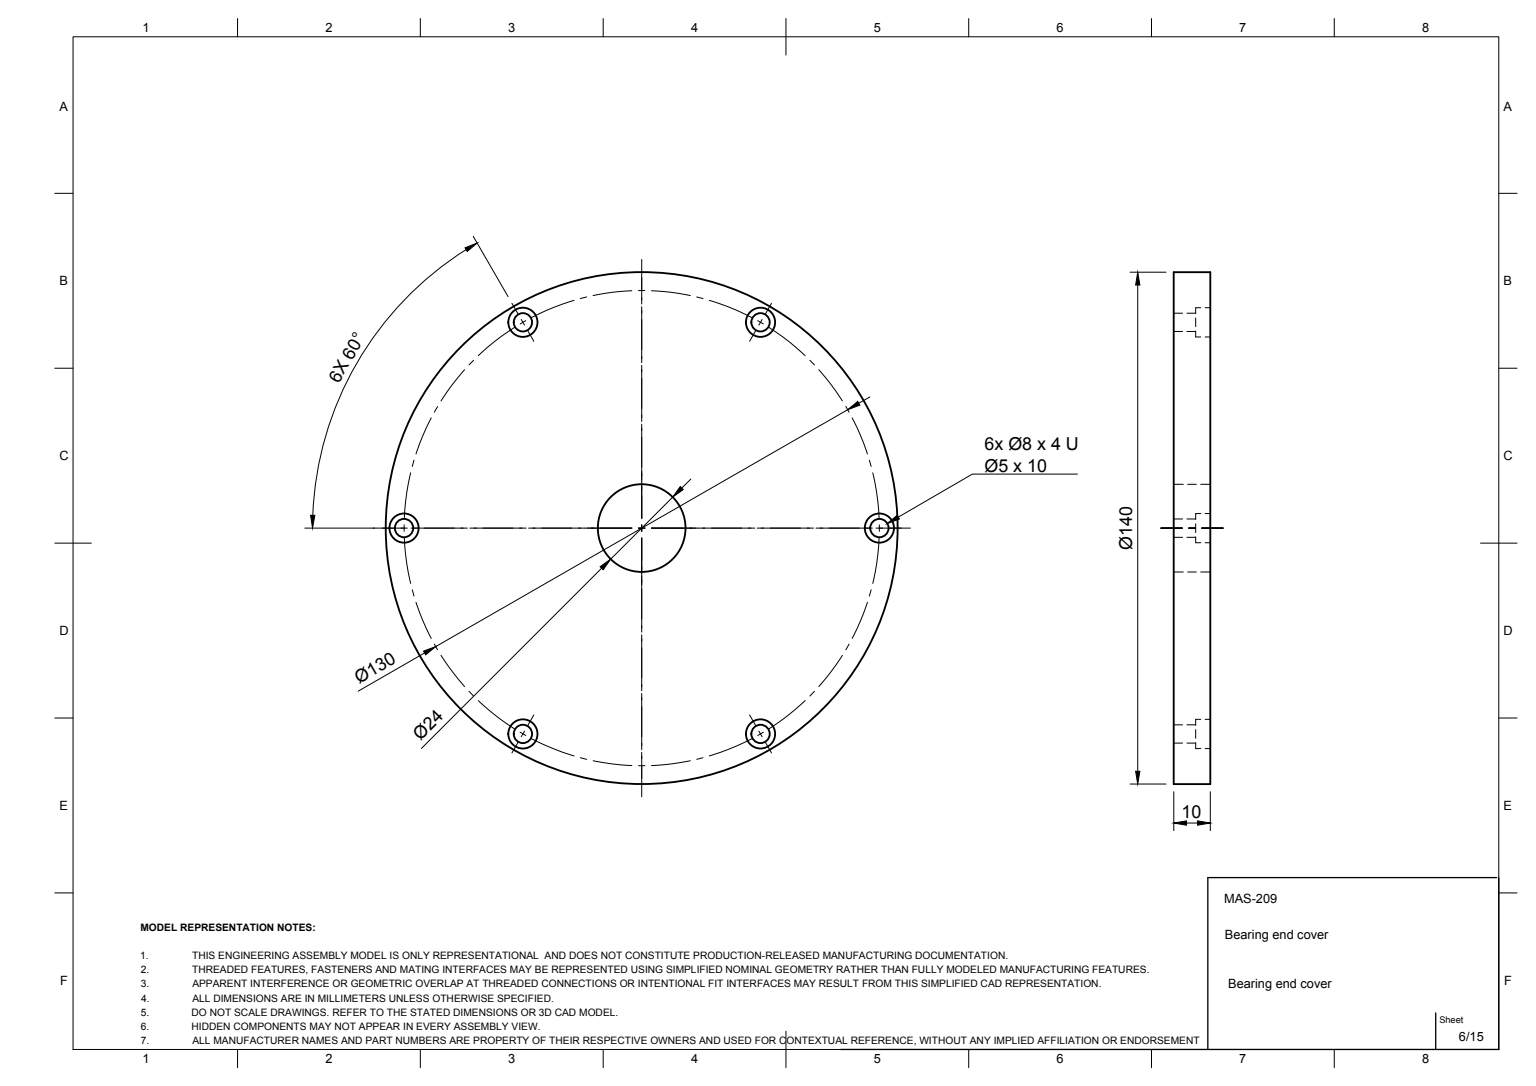
ISO-10303-21;
HEADER;
/* Generated by software containing ST-Developer
 * from STEP Tools, Inc. (www.steptools.com) 
 */

FILE_DESCRIPTION(
/* description */ ('Independent bearing-supported roller-ramp one-way clutch. Six logarit
hmic ramps with plain solid rollers, sprung guided plungers, native Co
il variants, removable shared keepers, rounded parallel key, shaft wit
h complete retaining lips, bronze journal/thrust support and bolted co
vers. Native rotor, roller planar/spin and plunger joints permit manua
l geometric engaged/released inspection. Automatic frictional torque s
witching/contact dynamics are not simulated; no capacity, hardness, fi
t, lubrication, speed, force or life rating. External input driver/cou
pling/anchors outside assembly.'),
/* implementation_level */ '2;1');

FILE_NAME(
/* name */ 'Bearing end cover.step',
/* time_stamp */ '2026-11-08T07:04:38-08:00',
/* author */ (''),
/* organization */ (''),
/* preprocessor_version */ 'ST-DEVELOPER v20.2',
/* originating_system */ 'Autodesk Translation Framework v15.17.0.0',
/* authorisation */ '');

FILE_SCHEMA (('AUTOMOTIVE_DESIGN { 1 0 10303 214 3 1 1 }'));
ENDSEC;

DATA;
#10=MECHANICAL_DESIGN_GEOMETRIC_PRESENTATION_REPRESENTATION('',(#305),#99526);
#273=SHAPE_REPRESENTATION_RELATIONSHIP('SRR','None',#99630,#289);
#289=ADVANCED_BREP_SHAPE_REPRESENTATION('',(#321),#99515);
#305=STYLED_ITEM('',(#99719),#321);
#321=MANIFOLD_SOLID_BREP('Body1',#18275);
#394=FACE_BOUND('',#2584,.T.);
#395=FACE_BOUND('',#2588,.T.);
#396=FACE_BOUND('',#2592,.T.);
#397=FACE_BOUND('',#2596,.T.);
#398=FACE_BOUND('',#2600,.T.);
#399=FACE_BOUND('',#2604,.T.);
#400=FACE_BOUND('',#2610,.T.);
#401=FACE_BOUND('',#2611,.T.);
#402=FACE_BOUND('',#2612,.T.);
#403=FACE_BOUND('',#2613,.T.);
#404=FACE_BOUND('',#2614,.T.);
#405=FACE_BOUND('',#2615,.T.);
#406=FACE_BOUND('',#2616,.T.);
#407=FACE_BOUND('',#2618,.T.);
#408=FACE_BOUND('',#2619,.T.);
#409=FACE_BOUND('',#2620,.T.);
#410=FACE_BOUND('',#2621,.T.);
#411=FACE_BOUND('',#2622,.T.);
#412=FACE_BOUND('',#2623,.T.);
#413=FACE_BOUND('',#2624,.T.);
#567=PLANE('',#19496);
#568=PLANE('',#19503);
#569=PLANE('',#19510);
#570=PLANE('',#19517);
#571=PLANE('',#19524);
#572=PLANE('',#19531);
#573=PLANE('',#19544);
#574=PLANE('',#19545);
#1524=FACE_OUTER_BOUND('',#2583,.T.);
#1525=FACE_OUTER_BOUND('',#2585,.T.);
#1526=FACE_OUTER_BOUND('',#2586,.T.);
#1527=FACE_OUTER_BOUND('',#2587,.T.);
#1528=FACE_OUTER_BOUND('',#2589,.T.);
#1529=FACE_OUTER_BOUND('',#2590,.T.);
#1530=FACE_OUTER_BOUND('',#2591,.T.);
#1531=FACE_OUTER_BOUND('',#2593,.T.);
#1532=FACE_OUTER_BOUND('',#2594,.T.);
#1533=FACE_OUTER_BOUND('',#2595,.T.);
#1534=FACE_OUTER_BOUND('',#2597,.T.);
#1535=FACE_OUTER_BOUND('',#2598,.T.);
#1536=FACE_OUTER_BOUND('',#2599,.T.);
#1537=FACE_OUTER_BOUND('',#2601,.T.);
#1538=FACE_OUTER_BOUND('',#2602,.T.);
#1539=FACE_OUTER_BOUND('',#2603,.T.);
#1540=FACE_OUTER_BOUND('',#2605,.T.);
#1541=FACE_OUTER_BOUND('',#2606,.T.);
#1542=FACE_OUTER_BOUND('',#2607,.T.);
#1543=FACE_OUTER_BOUND('',#2608,.T.);
#1544=FACE_OUTER_BOUND('',#2609,.T.);
#1545=FACE_OUTER_BOUND('',#2617,.T.);
#2583=EDGE_LOOP('',(#15852));
#2584=EDGE_LOOP('',(#15853));
#2585=EDGE_LOOP('',(#15854,#15855,#15856,#15857));
#2586=EDGE_LOOP('',(#15858,#15859,#15860,#15861));
#2587=EDGE_LOOP('',(#15862));
#2588=EDGE_LOOP('',(#15863));
#2589=EDGE_LOOP('',(#15864,#15865,#15866,#15867));
#2590=EDGE_LOOP('',(#15868,#15869,#15870,#15871));
#2591=EDGE_LOOP('',(#15872));
#2592=EDGE_LOOP('',(#15873));
#2593=EDGE_LOOP('',(#15874,#15875,#15876,#15877));
#2594=EDGE_LOOP('',(#15878,#15879,#15880,#15881));
#2595=EDGE_LOOP('',(#15882));
#2596=EDGE_LOOP('',(#15883));
#2597=EDGE_LOOP('',(#15884,#15885,#15886,#15887));
#2598=EDGE_LOOP('',(#15888,#15889,#15890,#15891));
#2599=EDGE_LOOP('',(#15892));
#2600=EDGE_LOOP('',(#15893));
#2601=EDGE_LOOP('',(#15894,#15895,#15896,#15897));
#2602=EDGE_LOOP('',(#15898,#15899,#15900,#15901));
#2603=EDGE_LOOP('',(#15902));
#2604=EDGE_LOOP('',(#15903));
#2605=EDGE_LOOP('',(#15904,#15905,#15906,#15907));
#2606=EDGE_LOOP('',(#15908,#15909,#15910,#15911));
#2607=EDGE_LOOP('',(#15912,#15913,#15914,#15915));
#2608=EDGE_LOOP('',(#15916,#15917,#15918,#15919));
#2609=EDGE_LOOP('',(#15920));
#2610=EDGE_LOOP('',(#15921));
#2611=EDGE_LOOP('',(#15922));
#2612=EDGE_LOOP('',(#15923));
#2613=EDGE_LOOP('',(#15924));
#2614=EDGE_LOOP('',(#15925));
#2615=EDGE_LOOP('',(#15926));
#2616=EDGE_LOOP('',(#15927));
#2617=EDGE_LOOP('',(#15928));
#2618=EDGE_LOOP('',(#15929));
#2619=EDGE_LOOP('',(#15930));
#2620=EDGE_LOOP('',(#15931));
#2621=EDGE_LOOP('',(#15932));
#2622=EDGE_LOOP('',(#15933));
#2623=EDGE_LOOP('',(#15934));
#2624=EDGE_LOOP('',(#15935));
#3022=CIRCLE('',#19497,4.);
#3023=CIRCLE('',#19498,2.5);
#3024=CIRCLE('',#19500,4.);
#3025=CIRCLE('',#19502,2.5);
#3026=CIRCLE('',#19504,4.);
#3027=CIRCLE('',#19505,2.5);
#3028=CIRCLE('',#19507,4.);
#3029=CIRCLE('',#19509,2.5);
#3030=CIRCLE('',#19511,4.);
#3031=CIRCLE('',#19512,2.5);
#3032=CIRCLE('',#19514,4.);
#3033=CIRCLE('',#19516,2.5);
#3034=CIRCLE('',#19518,4.);
#3035=CIRCLE('',#19519,2.5);
#3036=CIRCLE('',#19521,4.);
#3037=CIRCLE('',#19523,2.5);
#3038=CIRCLE('',#19525,4.);
#3039=CIRCLE('',#19526,2.5);
#3040=CIRCLE('',#19528,4.);
#3041=CIRCLE('',#19530,2.5);
#3042=CIRCLE('',#19532,4.);
#3043=CIRCLE('',#19533,2.5);
#3044=CIRCLE('',#19535,4.);
#3045=CIRCLE('',#19537,2.5);
#3046=CIRCLE('',#19539,12.);
#3047=CIRCLE('',#19540,12.);
#3048=CIRCLE('',#19542,70.);
#3049=CIRCLE('',#19543,70.);
#5400=LINE('',#94675,#6304);
#5401=LINE('',#94678,#6305);
#5402=LINE('',#94688,#6306);
#5403=LINE('',#94691,#6307);
#5404=LINE('',#94701,#6308);
#5405=LINE('',#94704,#6309);
#5406=LINE('',#94714,#6310);
#5407=LINE('',#94717,#6311);
#5408=LINE('',#94727,#6312);
#5409=LINE('',#94730,#6313);
#5410=LINE('',#94740,#6314);
#5411=LINE('',#94743,#6315);
#5412=LINE('',#94749,#6316);
#5413=LINE('',#94755,#6317);
#6304=VECTOR('',#22645,4.);
#6305=VECTOR('',#22648,2.5);
#6306=VECTOR('',#22661,4.);
#6307=VECTOR('',#22664,2.5);
#6308=VECTOR('',#22677,4.);
#6309=VECTOR('',#22680,2.5);
#6310=VECTOR('',#22693,4.);
#6311=VECTOR('',#22696,2.5);
#6312=VECTOR('',#22709,4.);
#6313=VECTOR('',#22712,2.5);
#6314=VECTOR('',#22725,4.);
#6315=VECTOR('',#22728,2.5);
#6316=VECTOR('',#22735,12.);
#6317=VECTOR('',#22742,70.);
#8037=VERTEX_POINT('',#94668);
#8038=VERTEX_POINT('',#94670);
#8039=VERTEX_POINT('',#94673);
#8040=VERTEX_POINT('',#94677);
#8041=VERTEX_POINT('',#94681);
#8042=VERTEX_POINT('',#94683);
#8043=VERTEX_POINT('',#94686);
#8044=VERTEX_POINT('',#94690);
#8045=VERTEX_POINT('',#94694);
#8046=VERTEX_POINT('',#94696);
#8047=VERTEX_POINT('',#94699);
#8048=VERTEX_POINT('',#94703);
#8049=VERTEX_POINT('',#94707);
#8050=VERTEX_POINT('',#94709);
#8051=VERTEX_POINT('',#94712);
#8052=VERTEX_POINT('',#94716);
#8053=VERTEX_POINT('',#94720);
#8054=VERTEX_POINT('',#94722);
#8055=VERTEX_POINT('',#94725);
#8056=VERTEX_POINT('',#94729);
#8057=VERTEX_POINT('',#94733);
#8058=VERTEX_POINT('',#94735);
#8059=VERTEX_POINT('',#94738);
#8060=VERTEX_POINT('',#94742);
#8061=VERTEX_POINT('',#94746);
#8062=VERTEX_POINT('',#94748);
#8063=VERTEX_POINT('',#94752);
#8064=VERTEX_POINT('',#94754);
#10678=EDGE_CURVE('',#8037,#8037,#3022,.T.);
#10679=EDGE_CURVE('',#8038,#8038,#3023,.T.);
#10680=EDGE_CURVE('',#8039,#8039,#3024,.T.);
#10681=EDGE_CURVE('',#8039,#8037,#5400,.T.);
#10682=EDGE_CURVE('',#8038,#8040,#5401,.T.);
#10683=EDGE_CURVE('',#8040,#8040,#3025,.T.);
#10684=EDGE_CURVE('',#8041,#8041,#3026,.T.);
#10685=EDGE_CURVE('',#8042,#8042,#3027,.T.);
#10686=EDGE_CURVE('',#8043,#8043,#3028,.T.);
#10687=EDGE_CURVE('',#8043,#8041,#5402,.T.);
#10688=EDGE_CURVE('',#8042,#8044,#5403,.T.);
#10689=EDGE_CURVE('',#8044,#8044,#3029,.T.);
#10690=EDGE_CURVE('',#8045,#8045,#3030,.T.);
#10691=EDGE_CURVE('',#8046,#8046,#3031,.T.);
#10692=EDGE_CURVE('',#8047,#8047,#3032,.T.);
#10693=EDGE_CURVE('',#8047,#8045,#5404,.T.);
#10694=EDGE_CURVE('',#8046,#8048,#5405,.T.);
#10695=EDGE_CURVE('',#8048,#8048,#3033,.T.);
#10696=EDGE_CURVE('',#8049,#8049,#3034,.T.);
#10697=EDGE_CURVE('',#8050,#8050,#3035,.T.);
#10698=EDGE_CURVE('',#8051,#8051,#3036,.T.);
#10699=EDGE_CURVE('',#8051,#8049,#5406,.T.);
#10700=EDGE_CURVE('',#8050,#8052,#5407,.T.);
#10701=EDGE_CURVE('',#8052,#8052,#3037,.T.);
#10702=EDGE_CURVE('',#8053,#8053,#3038,.T.);
#10703=EDGE_CURVE('',#8054,#8054,#3039,.T.);
#10704=EDGE_CURVE('',#8055,#8055,#3040,.T.);
#10705=EDGE_CURVE('',#8055,#8053,#5408,.T.);
#10706=EDGE_CURVE('',#8054,#8056,#5409,.T.);
#10707=EDGE_CURVE('',#8056,#8056,#3041,.T.);
#10708=EDGE_CURVE('',#8057,#8057,#3042,.T.);
#10709=EDGE_CURVE('',#8058,#8058,#3043,.T.);
#10710=EDGE_CURVE('',#8059,#8059,#3044,.T.);
#10711=EDGE_CURVE('',#8059,#8057,#5410,.T.);
#10712=EDGE_CURVE('',#8058,#8060,#5411,.T.);
#10713=EDGE_CURVE('',#8060,#8060,#3045,.T.);
#10714=EDGE_CURVE('',#8061,#8061,#3046,.T.);
#10715=EDGE_CURVE('',#8061,#8062,#5412,.T.);
#10716=EDGE_CURVE('',#8062,#8062,#3047,.T.);
#10717=EDGE_CURVE('',#8063,#8063,#3048,.T.);
#10718=EDGE_CURVE('',#8063,#8064,#5413,.T.);
#10719=EDGE_CURVE('',#8064,#8064,#3049,.T.);
#15852=ORIENTED_EDGE('',*,*,#10678,.F.);
#15853=ORIENTED_EDGE('',*,*,#10679,.T.);
#15854=ORIENTED_EDGE('',*,*,#10680,.F.);
#15855=ORIENTED_EDGE('',*,*,#10681,.T.);
#15856=ORIENTED_EDGE('',*,*,#10678,.T.);
#15857=ORIENTED_EDGE('',*,*,#10681,.F.);
#15858=ORIENTED_EDGE('',*,*,#10679,.F.);
#15859=ORIENTED_EDGE('',*,*,#10682,.T.);
#15860=ORIENTED_EDGE('',*,*,#10683,.F.);
#15861=ORIENTED_EDGE('',*,*,#10682,.F.);
#15862=ORIENTED_EDGE('',*,*,#10684,.F.);
#15863=ORIENTED_EDGE('',*,*,#10685,.T.);
#15864=ORIENTED_EDGE('',*,*,#10686,.F.);
#15865=ORIENTED_EDGE('',*,*,#10687,.T.);
#15866=ORIENTED_EDGE('',*,*,#10684,.T.);
#15867=ORIENTED_EDGE('',*,*,#10687,.F.);
#15868=ORIENTED_EDGE('',*,*,#10685,.F.);
#15869=ORIENTED_EDGE('',*,*,#10688,.T.);
#15870=ORIENTED_EDGE('',*,*,#10689,.F.);
#15871=ORIENTED_EDGE('',*,*,#10688,.F.);
#15872=ORIENTED_EDGE('',*,*,#10690,.F.);
#15873=ORIENTED_EDGE('',*,*,#10691,.T.);
#15874=ORIENTED_EDGE('',*,*,#10692,.F.);
#15875=ORIENTED_EDGE('',*,*,#10693,.T.);
#15876=ORIENTED_EDGE('',*,*,#10690,.T.);
#15877=ORIENTED_EDGE('',*,*,#10693,.F.);
#15878=ORIENTED_EDGE('',*,*,#10691,.F.);
#15879=ORIENTED_EDGE('',*,*,#10694,.T.);
#15880=ORIENTED_EDGE('',*,*,#10695,.F.);
#15881=ORIENTED_EDGE('',*,*,#10694,.F.);
#15882=ORIENTED_EDGE('',*,*,#10696,.F.);
#15883=ORIENTED_EDGE('',*,*,#10697,.T.);
#15884=ORIENTED_EDGE('',*,*,#10698,.F.);
#15885=ORIENTED_EDGE('',*,*,#10699,.T.);
#15886=ORIENTED_EDGE('',*,*,#10696,.T.);
#15887=ORIENTED_EDGE('',*,*,#10699,.F.);
#15888=ORIENTED_EDGE('',*,*,#10697,.F.);
#15889=ORIENTED_EDGE('',*,*,#10700,.T.);
#15890=ORIENTED_EDGE('',*,*,#10701,.F.);
#15891=ORIENTED_EDGE('',*,*,#10700,.F.);
#15892=ORIENTED_EDGE('',*,*,#10702,.F.);
#15893=ORIENTED_EDGE('',*,*,#10703,.T.);
#15894=ORIENTED_EDGE('',*,*,#10704,.F.);
#15895=ORIENTED_EDGE('',*,*,#10705,.T.);
#15896=ORIENTED_EDGE('',*,*,#10702,.T.);
#15897=ORIENTED_EDGE('',*,*,#10705,.F.);
#15898=ORIENTED_EDGE('',*,*,#10703,.F.);
#15899=ORIENTED_EDGE('',*,*,#10706,.T.);
#15900=ORIENTED_EDGE('',*,*,#10707,.F.);
#15901=ORIENTED_EDGE('',*,*,#10706,.F.);
#15902=ORIENTED_EDGE('',*,*,#10708,.F.);
#15903=ORIENTED_EDGE('',*,*,#10709,.T.);
#15904=ORIENTED_EDGE('',*,*,#10710,.F.);
#15905=ORIENTED_EDGE('',*,*,#10711,.T.);
#15906=ORIENTED_EDGE('',*,*,#10708,.T.);
#15907=ORIENTED_EDGE('',*,*,#10711,.F.);
#15908=ORIENTED_EDGE('',*,*,#10709,.F.);
#15909=ORIENTED_EDGE('',*,*,#10712,.T.);
#15910=ORIENTED_EDGE('',*,*,#10713,.F.);
#15911=ORIENTED_EDGE('',*,*,#10712,.F.);
#15912=ORIENTED_EDGE('',*,*,#10714,.F.);
#15913=ORIENTED_EDGE('',*,*,#10715,.T.);
#15914=ORIENTED_EDGE('',*,*,#10716,.T.);
#15915=ORIENTED_EDGE('',*,*,#10715,.F.);
#15916=ORIENTED_EDGE('',*,*,#10717,.F.);
#15917=ORIENTED_EDGE('',*,*,#10718,.T.);
#15918=ORIENTED_EDGE('',*,*,#10719,.T.);
#15919=ORIENTED_EDGE('',*,*,#10718,.F.);
#15920=ORIENTED_EDGE('',*,*,#10717,.T.);
#15921=ORIENTED_EDGE('',*,*,#10714,.T.);
#15922=ORIENTED_EDGE('',*,*,#10710,.T.);
#15923=ORIENTED_EDGE('',*,*,#10704,.T.);
#15924=ORIENTED_EDGE('',*,*,#10698,.T.);
#15925=ORIENTED_EDGE('',*,*,#10692,.T.);
#15926=ORIENTED_EDGE('',*,*,#10686,.T.);
#15927=ORIENTED_EDGE('',*,*,#10680,.T.);
#15928=ORIENTED_EDGE('',*,*,#10719,.F.);
#15929=ORIENTED_EDGE('',*,*,#10716,.F.);
#15930=ORIENTED_EDGE('',*,*,#10713,.T.);
#15931=ORIENTED_EDGE('',*,*,#10707,.T.);
#15932=ORIENTED_EDGE('',*,*,#10701,.T.);
#15933=ORIENTED_EDGE('',*,*,#10695,.T.);
#15934=ORIENTED_EDGE('',*,*,#10689,.T.);
#15935=ORIENTED_EDGE('',*,*,#10683,.T.);
#17186=CYLINDRICAL_SURFACE('',#19499,4.);
#17187=CYLINDRICAL_SURFACE('',#19501,2.5);
#17188=CYLINDRICAL_SURFACE('',#19506,4.);
#17189=CYLINDRICAL_SURFACE('',#19508,2.5);
#17190=CYLINDRICAL_SURFACE('',#19513,4.);
#17191=CYLINDRICAL_SURFACE('',#19515,2.5);
#17192=CYLINDRICAL_SURFACE('',#19520,4.);
#17193=CYLINDRICAL_SURFACE('',#19522,2.5);
#17194=CYLINDRICAL_SURFACE('',#19527,4.);
#17195=CYLINDRICAL_SURFACE('',#19529,2.5);
#17196=CYLINDRICAL_SURFACE('',#19534,4.);
#17197=CYLINDRICAL_SURFACE('',#19536,2.5);
#17198=CYLINDRICAL_SURFACE('',#19538,12.);
#17199=CYLINDRICAL_SURFACE('',#19541,70.);
#18122=ADVANCED_FACE('',(#1524,#394),#567,.F.);
#18123=ADVANCED_FACE('',(#1525),#17186,.F.);
#18124=ADVANCED_FACE('',(#1526),#17187,.F.);
#18125=ADVANCED_FACE('',(#1527,#395),#568,.F.);
#18126=ADVANCED_FACE('',(#1528),#17188,.F.);
#18127=ADVANCED_FACE('',(#1529),#17189,.F.);
#18128=ADVANCED_FACE('',(#1530,#396),#569,.F.);
#18129=ADVANCED_FACE('',(#1531),#17190,.F.);
#18130=ADVANCED_FACE('',(#1532),#17191,.F.);
#18131=ADVANCED_FACE('',(#1533,#397),#570,.F.);
#18132=ADVANCED_FACE('',(#1534),#17192,.F.);
#18133=ADVANCED_FACE('',(#1535),#17193,.F.);
#18134=ADVANCED_FACE('',(#1536,#398),#571,.F.);
#18135=ADVANCED_FACE('',(#1537),#17194,.F.);
#18136=ADVANCED_FACE('',(#1538),#17195,.F.);
#18137=ADVANCED_FACE('',(#1539,#399),#572,.F.);
#18138=ADVANCED_FACE('',(#1540),#17196,.F.);
#18139=ADVANCED_FACE('',(#1541),#17197,.F.);
#18140=ADVANCED_FACE('',(#1542),#17198,.F.);
#18141=ADVANCED_FACE('',(#1543),#17199,.T.);
#18142=ADVANCED_FACE('',(#1544,#400,#401,#402,#403,#404,#405,#406),#573,
 .T.);
#18143=ADVANCED_FACE('',(#1545,#407,#408,#409,#410,#411,#412,#413),#574,
 .F.);
#18275=CLOSED_SHELL('',(#18122,#18123,#18124,#18125,#18126,#18127,#18128,
#18129,#18130,#18131,#18132,#18133,#18134,#18135,#18136,#18137,#18138,#18139,
#18140,#18141,#18142,#18143));
#19495=AXIS2_PLACEMENT_3D('',#94666,#22633,#22634);
#19496=AXIS2_PLACEMENT_3D('',#94667,#22635,#22636);
#19497=AXIS2_PLACEMENT_3D('',#94669,#22637,#22638);
#19498=AXIS2_PLACEMENT_3D('',#94671,#22639,#22640);
#19499=AXIS2_PLACEMENT_3D('',#94672,#22641,#22642);
#19500=AXIS2_PLACEMENT_3D('',#94674,#22643,#22644);
#19501=AXIS2_PLACEMENT_3D('',#94676,#22646,#22647);
#19502=AXIS2_PLACEMENT_3D('',#94679,#22649,#22650);
#19503=AXIS2_PLACEMENT_3D('',#94680,#22651,#22652);
#19504=AXIS2_PLACEMENT_3D('',#94682,#22653,#22654);
#19505=AXIS2_PLACEMENT_3D('',#94684,#22655,#22656);
#19506=AXIS2_PLACEMENT_3D('',#94685,#22657,#22658);
#19507=AXIS2_PLACEMENT_3D('',#94687,#22659,#22660);
#19508=AXIS2_PLACEMENT_3D('',#94689,#22662,#22663);
#19509=AXIS2_PLACEMENT_3D('',#94692,#22665,#22666);
#19510=AXIS2_PLACEMENT_3D('',#94693,#22667,#22668);
#19511=AXIS2_PLACEMENT_3D('',#94695,#22669,#22670);
#19512=AXIS2_PLACEMENT_3D('',#94697,#22671,#22672);
#19513=AXIS2_PLACEMENT_3D('',#94698,#22673,#22674);
#19514=AXIS2_PLACEMENT_3D('',#94700,#22675,#22676);
#19515=AXIS2_PLACEMENT_3D('',#94702,#22678,#22679);
#19516=AXIS2_PLACEMENT_3D('',#94705,#22681,#22682);
#19517=AXIS2_PLACEMENT_3D('',#94706,#22683,#22684);
#19518=AXIS2_PLACEMENT_3D('',#94708,#22685,#22686);
#19519=AXIS2_PLACEMENT_3D('',#94710,#22687,#22688);
#19520=AXIS2_PLACEMENT_3D('',#94711,#22689,#22690);
#19521=AXIS2_PLACEMENT_3D('',#94713,#22691,#22692);
#19522=AXIS2_PLACEMENT_3D('',#94715,#22694,#22695);
#19523=AXIS2_PLACEMENT_3D('',#94718,#22697,#22698);
#19524=AXIS2_PLACEMENT_3D('',#94719,#22699,#22700);
#19525=AXIS2_PLACEMENT_3D('',#94721,#22701,#22702);
#19526=AXIS2_PLACEMENT_3D('',#94723,#22703,#22704);
#19527=AXIS2_PLACEMENT_3D('',#94724,#22705,#22706);
#19528=AXIS2_PLACEMENT_3D('',#94726,#22707,#22708);
#19529=AXIS2_PLACEMENT_3D('',#94728,#22710,#22711);
#19530=AXIS2_PLACEMENT_3D('',#94731,#22713,#22714);
#19531=AXIS2_PLACEMENT_3D('',#94732,#22715,#22716);
#19532=AXIS2_PLACEMENT_3D('',#94734,#22717,#22718);
#19533=AXIS2_PLACEMENT_3D('',#94736,#22719,#22720);
#19534=AXIS2_PLACEMENT_3D('',#94737,#22721,#22722);
#19535=AXIS2_PLACEMENT_3D('',#94739,#22723,#22724);
#19536=AXIS2_PLACEMENT_3D('',#94741,#22726,#22727);
#19537=AXIS2_PLACEMENT_3D('',#94744,#22729,#22730);
#19538=AXIS2_PLACEMENT_3D('',#94745,#22731,#22732);
#19539=AXIS2_PLACEMENT_3D('',#94747,#22733,#22734);
#19540=AXIS2_PLACEMENT_3D('',#94750,#22736,#22737);
#19541=AXIS2_PLACEMENT_3D('',#94751,#22738,#22739);
#19542=AXIS2_PLACEMENT_3D('',#94753,#22740,#22741);
#19543=AXIS2_PLACEMENT_3D('',#94756,#22743,#22744);
#19544=AXIS2_PLACEMENT_3D('',#94757,#22745,#22746);
#19545=AXIS2_PLACEMENT_3D('',#94758,#22747,#22748);
#22633=DIRECTION('axis',(0.,0.,1.));
#22634=DIRECTION('refdir',(1.,0.,0.));
#22635=DIRECTION('center_axis',(0.,0.,-1.));
#22636=DIRECTION('ref_axis',(1.,0.,0.));
#22637=DIRECTION('center_axis',(0.,0.,-1.));
#22638=DIRECTION('ref_axis',(1.,0.,0.));
#22639=DIRECTION('center_axis',(0.,0.,-1.));
#22640=DIRECTION('ref_axis',(1.,0.,0.));
#22641=DIRECTION('center_axis',(0.,0.,-1.));
#22642=DIRECTION('ref_axis',(1.,0.,0.));
#22643=DIRECTION('center_axis',(0.,0.,-1.));
#22644=DIRECTION('ref_axis',(1.,0.,0.));
#22645=DIRECTION('',(0.,0.,-1.));
#22646=DIRECTION('center_axis',(0.,0.,-1.));
#22647=DIRECTION('ref_axis',(1.,0.,0.));
#22648=DIRECTION('',(0.,0.,-1.));
#22649=DIRECTION('center_axis',(0.,0.,1.));
#22650=DIRECTION('ref_axis',(1.,0.,0.));
#22651=DIRECTION('center_axis',(0.,0.,-1.));
#22652=DIRECTION('ref_axis',(1.,0.,0.));
#22653=DIRECTION('center_axis',(0.,0.,-1.));
#22654=DIRECTION('ref_axis',(1.,0.,0.));
#22655=DIRECTION('center_axis',(0.,0.,-1.));
#22656=DIRECTION('ref_axis',(1.,0.,0.));
#22657=DIRECTION('center_axis',(0.,0.,-1.));
#22658=DIRECTION('ref_axis',(1.,0.,0.));
#22659=DIRECTION('center_axis',(0.,0.,-1.));
#22660=DIRECTION('ref_axis',(1.,0.,0.));
#22661=DIRECTION('',(0.,0.,-1.));
#22662=DIRECTION('center_axis',(0.,0.,-1.));
#22663=DIRECTION('ref_axis',(1.,0.,0.));
#22664=DIRECTION('',(0.,0.,-1.));
#22665=DIRECTION('center_axis',(0.,0.,1.));
#22666=DIRECTION('ref_axis',(1.,0.,0.));
#22667=DIRECTION('center_axis',(0.,0.,-1.));
#22668=DIRECTION('ref_axis',(1.,0.,0.));
#22669=DIRECTION('center_axis',(0.,0.,-1.));
#22670=DIRECTION('ref_axis',(1.,0.,0.));
#22671=DIRECTION('center_axis',(0.,0.,-1.));
#22672=DIRECTION('ref_axis',(1.,0.,0.));
#22673=DIRECTION('center_axis',(0.,0.,-1.));
#22674=DIRECTION('ref_axis',(1.,0.,0.));
#22675=DIRECTION('center_axis',(0.,0.,-1.));
#22676=DIRECTION('ref_axis',(1.,0.,0.));
#22677=DIRECTION('',(0.,0.,-1.));
#22678=DIRECTION('center_axis',(0.,0.,-1.));
#22679=DIRECTION('ref_axis',(1.,0.,0.));
#22680=DIRECTION('',(0.,0.,-1.));
#22681=DIRECTION('center_axis',(0.,0.,1.));
#22682=DIRECTION('ref_axis',(1.,0.,0.));
#22683=DIRECTION('center_axis',(0.,0.,-1.));
#22684=DIRECTION('ref_axis',(1.,0.,0.));
#22685=DIRECTION('center_axis',(0.,0.,-1.));
#22686=DIRECTION('ref_axis',(1.,0.,0.));
#22687=DIRECTION('center_axis',(0.,0.,-1.));
#22688=DIRECTION('ref_axis',(1.,0.,0.));
#22689=DIRECTION('center_axis',(0.,0.,-1.));
#22690=DIRECTION('ref_axis',(1.,0.,0.));
#22691=DIRECTION('center_axis',(0.,0.,-1.));
#22692=DIRECTION('ref_axis',(1.,0.,0.));
#22693=DIRECTION('',(0.,0.,-1.));
#22694=DIRECTION('center_axis',(0.,0.,-1.));
#22695=DIRECTION('ref_axis',(1.,0.,0.));
#22696=DIRECTION('',(0.,0.,-1.));
#22697=DIRECTION('center_axis',(0.,0.,1.));
#22698=DIRECTION('ref_axis',(1.,0.,0.));
#22699=DIRECTION('center_axis',(0.,0.,-1.));
#22700=DIRECTION('ref_axis',(1.,0.,0.));
#22701=DIRECTION('center_axis',(0.,0.,-1.));
#22702=DIRECTION('ref_axis',(1.,0.,0.));
#22703=DIRECTION('center_axis',(0.,0.,-1.));
#22704=DIRECTION('ref_axis',(1.,0.,0.));
#22705=DIRECTION('center_axis',(0.,0.,-1.));
#22706=DIRECTION('ref_axis',(1.,0.,0.));
#22707=DIRECTION('center_axis',(0.,0.,-1.));
#22708=DIRECTION('ref_axis',(1.,0.,0.));
#22709=DIRECTION('',(0.,0.,-1.));
#22710=DIRECTION('center_axis',(0.,0.,-1.));
#22711=DIRECTION('ref_axis',(1.,0.,0.));
#22712=DIRECTION('',(0.,0.,-1.));
#22713=DIRECTION('center_axis',(0.,0.,1.));
#22714=DIRECTION('ref_axis',(1.,0.,0.));
#22715=DIRECTION('center_axis',(0.,0.,-1.));
#22716=DIRECTION('ref_axis',(1.,0.,0.));
#22717=DIRECTION('center_axis',(0.,0.,-1.));
#22718=DIRECTION('ref_axis',(1.,0.,0.));
#22719=DIRECTION('center_axis',(0.,0.,-1.));
#22720=DIRECTION('ref_axis',(1.,0.,0.));
#22721=DIRECTION('center_axis',(0.,0.,-1.));
#22722=DIRECTION('ref_axis',(1.,0.,0.));
#22723=DIRECTION('center_axis',(0.,0.,-1.));
#22724=DIRECTION('ref_axis',(1.,0.,0.));
#22725=DIRECTION('',(0.,0.,-1.));
#22726=DIRECTION('center_axis',(0.,0.,-1.));
#22727=DIRECTION('ref_axis',(1.,0.,0.));
#22728=DIRECTION('',(0.,0.,-1.));
#22729=DIRECTION('center_axis',(0.,0.,1.));
#22730=DIRECTION('ref_axis',(1.,0.,0.));
#22731=DIRECTION('center_axis',(0.,0.,1.));
#22732=DIRECTION('ref_axis',(1.,0.,0.));
#22733=DIRECTION('center_axis',(0.,0.,-1.));
#22734=DIRECTION('ref_axis',(1.,0.,0.));
#22735=DIRECTION('',(0.,0.,-1.));
#22736=DIRECTION('center_axis',(0.,0.,-1.));
#22737=DIRECTION('ref_axis',(1.,0.,0.));
#22738=DIRECTION('center_axis',(0.,0.,1.));
#22739=DIRECTION('ref_axis',(1.,0.,0.));
#22740=DIRECTION('center_axis',(0.,0.,1.));
#22741=DIRECTION('ref_axis',(1.,0.,0.));
#22742=DIRECTION('',(0.,0.,-1.));
#22743=DIRECTION('center_axis',(0.,0.,1.));
#22744=DIRECTION('ref_axis',(1.,0.,0.));
#22745=DIRECTION('center_axis',(0.,0.,1.));
#22746=DIRECTION('ref_axis',(1.,0.,0.));
#22747=DIRECTION('center_axis',(0.,0.,1.));
#22748=DIRECTION('ref_axis',(1.,0.,0.));
#94666=CARTESIAN_POINT('',(0.,0.,0.));
#94667=CARTESIAN_POINT('Origin',(-32.5,-56.2916512459885,6.));
#94668=CARTESIAN_POINT('',(-36.5,-56.2916512459885,6.));
#94669=CARTESIAN_POINT('Origin',(-32.5,-56.2916512459885,6.));
#94670=CARTESIAN_POINT('',(-35.,-56.2916512459885,6.));
#94671=CARTESIAN_POINT('Origin',(-32.5,-56.2916512459885,6.));
#94672=CARTESIAN_POINT('Origin',(-32.5,-56.2916512459885,8.));
#94673=CARTESIAN_POINT('',(-36.5,-56.2916512459885,10.));
#94674=CARTESIAN_POINT('Origin',(-32.5,-56.2916512459885,10.));
#94675=CARTESIAN_POINT('',(-36.5,-56.2916512459885,8.));
#94676=CARTESIAN_POINT('Origin',(-32.5,-56.2916512459885,5.));
#94677=CARTESIAN_POINT('',(-35.,-56.2916512459885,0.));
#94678=CARTESIAN_POINT('',(-35.,-56.2916512459885,5.));
#94679=CARTESIAN_POINT('Origin',(-32.5,-56.2916512459885,0.));
#94680=CARTESIAN_POINT('Origin',(-32.5,56.2916512459885,6.));
#94681=CARTESIAN_POINT('',(-36.5,56.2916512459885,6.));
#94682=CARTESIAN_POINT('Origin',(-32.5,56.2916512459885,6.));
#94683=CARTESIAN_POINT('',(-35.,56.2916512459885,6.));
#94684=CARTESIAN_POINT('Origin',(-32.5,56.2916512459885,6.));
#94685=CARTESIAN_POINT('Origin',(-32.5,56.2916512459885,8.));
#94686=CARTESIAN_POINT('',(-36.5,56.2916512459885,10.));
#94687=CARTESIAN_POINT('Origin',(-32.5,56.2916512459885,10.));
#94688=CARTESIAN_POINT('',(-36.5,56.2916512459885,8.));
#94689=CARTESIAN_POINT('Origin',(-32.5,56.2916512459885,5.));
#94690=CARTESIAN_POINT('',(-35.,56.2916512459885,0.));
#94691=CARTESIAN_POINT('',(-35.,56.2916512459885,5.));
#94692=CARTESIAN_POINT('Origin',(-32.5,56.2916512459885,0.));
#94693=CARTESIAN_POINT('Origin',(65.,0.,6.));
#94694=CARTESIAN_POINT('',(61.,4.89858719658941E-16,6.));
#94695=CARTESIAN_POINT('Origin',(65.,0.,6.));
#94696=CARTESIAN_POINT('',(62.5,3.06161699786838E-16,6.));
#94697=CARTESIAN_POINT('Origin',(65.,0.,6.));
#94698=CARTESIAN_POINT('Origin',(65.,0.,8.));
#94699=CARTESIAN_POINT('',(61.,4.89858719658941E-16,10.));
#94700=CARTESIAN_POINT('Origin',(65.,0.,10.));
#94701=CARTESIAN_POINT('',(61.,4.89858719658941E-16,8.));
#94702=CARTESIAN_POINT('Origin',(65.,0.,5.));
#94703=CARTESIAN_POINT('',(62.5,3.06161699786838E-16,0.));
#94704=CARTESIAN_POINT('',(62.5,3.06161699786838E-16,5.));
#94705=CARTESIAN_POINT('Origin',(65.,0.,0.));
#94706=CARTESIAN_POINT('Origin',(32.5,56.2916512459885,6.));
#94707=CARTESIAN_POINT('',(28.5,56.2916512459885,6.));
#94708=CARTESIAN_POINT('Origin',(32.5,56.2916512459885,6.));
#94709=CARTESIAN_POINT('',(30.,56.2916512459885,6.));
#94710=CARTESIAN_POINT('Origin',(32.5,56.2916512459885,6.));
#94711=CARTESIAN_POINT('Origin',(32.5,56.2916512459885,8.));
#94712=CARTESIAN_POINT('',(28.5,56.2916512459885,10.));
#94713=CARTESIAN_POINT('Origin',(32.5,56.2916512459885,10.));
#94714=CARTESIAN_POINT('',(28.5,56.2916512459885,8.));
#94715=CARTESIAN_POINT('Origin',(32.5,56.2916512459885,5.));
#94716=CARTESIAN_POINT('',(30.,56.2916512459885,0.));
#94717=CARTESIAN_POINT('',(30.,56.2916512459885,5.));
#94718=CARTESIAN_POINT('Origin',(32.5,56.2916512459885,0.));
#94719=CARTESIAN_POINT('Origin',(-65.,7.9602041944578E-15,6.));
#94720=CARTESIAN_POINT('',(-69.,8.45006291411674E-15,6.));
#94721=CARTESIAN_POINT('Origin',(-65.,7.9602041944578E-15,6.));
#94722=CARTESIAN_POINT('',(-67.5,8.26636589424463E-15,6.));
#94723=CARTESIAN_POINT('Origin',(-65.,7.9602041944578E-15,6.));
#94724=CARTESIAN_POINT('Origin',(-65.,7.9602041944578E-15,8.));
#94725=CARTESIAN_POINT('',(-69.,8.45006291411674E-15,10.));
#94726=CARTESIAN_POINT('Origin',(-65.,7.9602041944578E-15,10.));
#94727=CARTESIAN_POINT('',(-69.,8.45006291411674E-15,8.));
#94728=CARTESIAN_POINT('Origin',(-65.,7.9602041944578E-15,5.));
#94729=CARTESIAN_POINT('',(-67.5,8.26636589424463E-15,0.));
#94730=CARTESIAN_POINT('',(-67.5,8.26636589424463E-15,5.));
#94731=CARTESIAN_POINT('Origin',(-65.,7.9602041944578E-15,0.));
#94732=CARTESIAN_POINT('Origin',(32.5,-56.2916512459885,6.));
#94733=CARTESIAN_POINT('',(28.5,-56.2916512459885,6.));
#94734=CARTESIAN_POINT('Origin',(32.5,-56.2916512459885,6.));
#94735=CARTESIAN_POINT('',(30.,-56.2916512459885,6.));
#94736=CARTESIAN_POINT('Origin',(32.5,-56.2916512459885,6.));
#94737=CARTESIAN_POINT('Origin',(32.5,-56.2916512459885,8.));
#94738=CARTESIAN_POINT('',(28.5,-56.2916512459885,10.));
#94739=CARTESIAN_POINT('Origin',(32.5,-56.2916512459885,10.));
#94740=CARTESIAN_POINT('',(28.5,-56.2916512459885,8.));
#94741=CARTESIAN_POINT('Origin',(32.5,-56.2916512459885,5.));
#94742=CARTESIAN_POINT('',(30.,-56.2916512459885,0.));
#94743=CARTESIAN_POINT('',(30.,-56.2916512459885,5.));
#94744=CARTESIAN_POINT('Origin',(32.5,-56.2916512459885,0.));
#94745=CARTESIAN_POINT('Origin',(0.,0.,0.));
#94746=CARTESIAN_POINT('',(-12.,-1.46957615897682E-15,10.));
#94747=CARTESIAN_POINT('Origin',(0.,0.,10.));
#94748=CARTESIAN_POINT('',(-12.,-1.46957615897682E-15,0.));
#94749=CARTESIAN_POINT('',(-12.,-1.46957615897682E-15,0.));
#94750=CARTESIAN_POINT('Origin',(0.,0.,0.));
#94751=CARTESIAN_POINT('Origin',(0.,0.,0.));
#94752=CARTESIAN_POINT('',(-70.,-8.57252759403147E-15,10.));
#94753=CARTESIAN_POINT('Origin',(0.,0.,10.));
#94754=CARTESIAN_POINT('',(-70.,-8.57252759403147E-15,0.));
#94755=CARTESIAN_POINT('',(-70.,-8.57252759403147E-15,0.));
#94756=CARTESIAN_POINT('Origin',(0.,0.,0.));
#94757=CARTESIAN_POINT('Origin',(0.,0.,10.));
#94758=CARTESIAN_POINT('Origin',(0.,0.,0.));
#99497=UNCERTAINTY_MEASURE_WITH_UNIT(LENGTH_MEASURE(0.01),#99527,
'DISTANCE_ACCURACY_VALUE',
'Maximum model space distance between geometric entities at asserted c
onnectivities');
#99508=UNCERTAINTY_MEASURE_WITH_UNIT(LENGTH_MEASURE(0.01),#99527,
'DISTANCE_ACCURACY_VALUE',
'Maximum model space distance between geometric entities at asserted c
onnectivities');
#99515=(
GEOMETRIC_REPRESENTATION_CONTEXT(3)
GLOBAL_UNCERTAINTY_ASSIGNED_CONTEXT((#99497))
GLOBAL_UNIT_ASSIGNED_CONTEXT((#99527,#99529,#99530))
REPRESENTATION_CONTEXT('','3D')
);
#99526=(
GEOMETRIC_REPRESENTATION_CONTEXT(3)
GLOBAL_UNCERTAINTY_ASSIGNED_CONTEXT((#99508))
GLOBAL_UNIT_ASSIGNED_CONTEXT((#99527,#99529,#99530))
REPRESENTATION_CONTEXT('','3D')
);
#99527=(
LENGTH_UNIT()
NAMED_UNIT(*)
SI_UNIT(.MILLI.,.METRE.)
);
#99529=(
NAMED_UNIT(*)
PLANE_ANGLE_UNIT()
SI_UNIT($,.RADIAN.)
);
#99530=(
NAMED_UNIT(*)
SI_UNIT($,.STERADIAN.)
SOLID_ANGLE_UNIT()
);
#99537=SHAPE_DEFINITION_REPRESENTATION(#99554,#99630);
#99554=PRODUCT_DEFINITION_SHAPE('',$,#99648);
#99630=SHAPE_REPRESENTATION('',(#19495),#99515);
#99641=PRODUCT_DEFINITION_CONTEXT('part definition',#99694,'design');
#99648=PRODUCT_DEFINITION('Bearing end cover','Bearing end cover',#99665,
#99641);
#99665=PRODUCT_DEFINITION_FORMATION('',$,#99702);
#99694=APPLICATION_CONTEXT(
'Core Data for Automotive Mechanical Design Process');
#99695=PRODUCT_CONTEXT('part definition',#99694,'mechanical');
#99702=PRODUCT('Bearing end cover','Bearing end cover',$,(#99695));
#99719=PRESENTATION_STYLE_ASSIGNMENT((#99732));
#99732=SURFACE_STYLE_USAGE(.BOTH.,#99745);
#99745=SURFACE_SIDE_STYLE('',(#99758));
#99758=SURFACE_STYLE_FILL_AREA(#99771);
#99771=FILL_AREA_STYLE('Sky blue',(#99784));
#99784=FILL_AREA_STYLE_COLOUR('Sky blue',#99797);
#99797=COLOUR_RGB('Sky blue',0.317647058823529,0.686274509803922,0.890196078431372);
ENDSEC;
END-ISO-10303-21;
